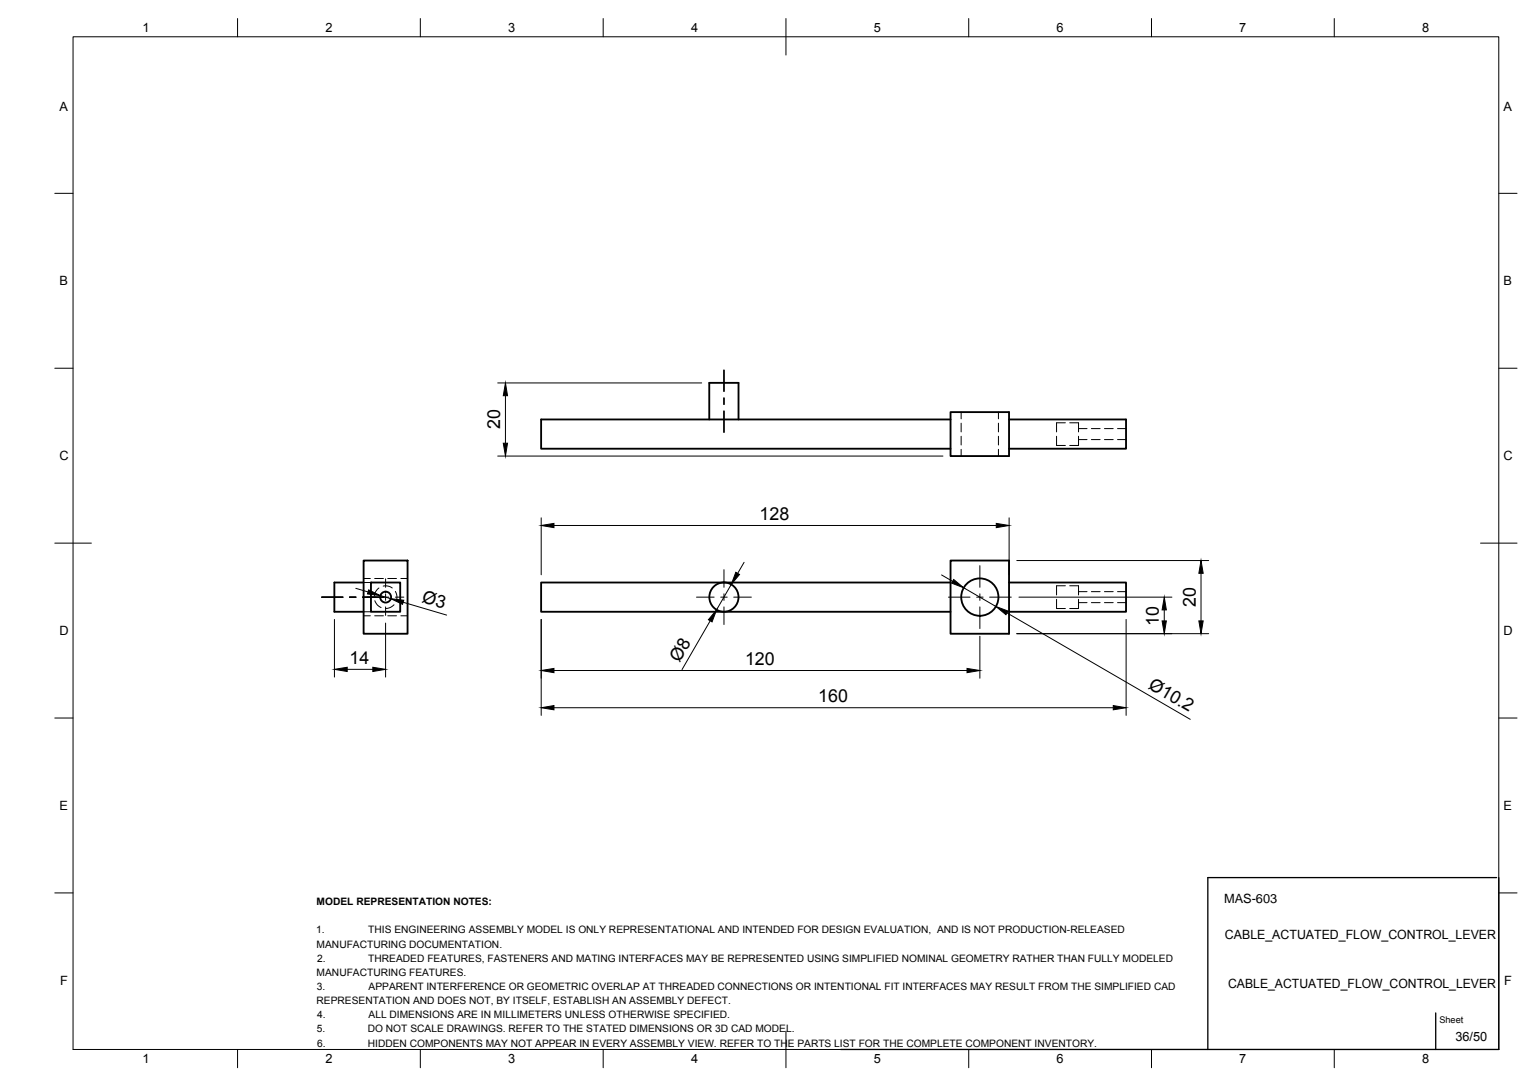
ISO-10303-21;
HEADER;
FILE_DESCRIPTION((''),'2;1');
FILE_NAME('CABLE_ACTUATED_FLOW_CONTROL_LEVER.step','2026-10-01T22:06:14-07:00',(''),(''),'','','');
FILE_SCHEMA (('AUTOMOTIVE_DESIGN { 1 0 10303 214 3 1 1 }'));
ENDSEC;
DATA;
#10=MECHANICAL_DESIGN_GEOMETRIC_PRESENTATION_REPRESENTATION('',(#1009),#50440);
#916=SHAPE_REPRESENTATION_RELATIONSHIP('SRR','None',#50649,#961) ;
#961=ADVANCED_BREP_SHAPE_REPRESENTATION('',(#1064),#50418) ;
#1009=STYLED_ITEM('',(#50883),#1064) ;
#1064=MANIFOLD_SOLID_BREP('CABLE_ACTUATED_FLOW_CONTROL_LEVER',#28676) ;
#1370=FACE_BOUND('',#5206,.T.) ;
#1371=FACE_BOUND('',#5211,.T.) ;
#1372=FACE_BOUND('',#5213,.T.) ;
#1373=FACE_BOUND('',#5215,.T.) ;
#1374=FACE_BOUND('',#5218,.T.) ;
#1375=FACE_BOUND('',#5229,.T.) ;
#2208=PLANE('',#30896) ;
#2209=PLANE('',#30897) ;
#2210=PLANE('',#30898) ;
#2211=PLANE('',#30902) ;
#2212=PLANE('',#30904) ;
#2213=PLANE('',#30910) ;
#2214=PLANE('',#30911) ;
#2215=PLANE('',#30912) ;
#2216=PLANE('',#30913) ;
#2217=PLANE('',#30914) ;
#2218=PLANE('',#30915) ;
#2219=PLANE('',#30916) ;
#2220=PLANE('',#30917) ;
#2221=PLANE('',#30918) ;
#2222=PLANE('',#30919) ;
#2223=PLANE('',#30920) ;
#2224=PLANE('',#30921) ;
#2225=PLANE('',#30922) ;
#2226=PLANE('',#30923) ;
#2227=PLANE('',#30924) ;
#3388=FACE_OUTER_BOUND('',#5200,.T.) ;
#3389=FACE_OUTER_BOUND('',#5201,.T.) ;
#3390=FACE_OUTER_BOUND('',#5202,.T.) ;
#3391=FACE_OUTER_BOUND('',#5203,.T.) ;
#3392=FACE_OUTER_BOUND('',#5204,.T.) ;
#3393=FACE_OUTER_BOUND('',#5205,.T.) ;
#3394=FACE_OUTER_BOUND('',#5207,.T.) ;
#3395=FACE_OUTER_BOUND('',#5208,.T.) ;
#3396=FACE_OUTER_BOUND('',#5209,.T.) ;
#3397=FACE_OUTER_BOUND('',#5210,.T.) ;
#3398=FACE_OUTER_BOUND('',#5212,.T.) ;
#3399=FACE_OUTER_BOUND('',#5214,.T.) ;
#3400=FACE_OUTER_BOUND('',#5216,.T.) ;
#3401=FACE_OUTER_BOUND('',#5217,.T.) ;
#3402=FACE_OUTER_BOUND('',#5219,.T.) ;
#3403=FACE_OUTER_BOUND('',#5220,.T.) ;
#3404=FACE_OUTER_BOUND('',#5221,.T.) ;
#3405=FACE_OUTER_BOUND('',#5222,.T.) ;
#3406=FACE_OUTER_BOUND('',#5223,.T.) ;
#3407=FACE_OUTER_BOUND('',#5224,.T.) ;
#3408=FACE_OUTER_BOUND('',#5225,.T.) ;
#3409=FACE_OUTER_BOUND('',#5226,.T.) ;
#3410=FACE_OUTER_BOUND('',#5227,.T.) ;
#3411=FACE_OUTER_BOUND('',#5228,.T.) ;
#5200=EDGE_LOOP('',(#23983,#23984,#23985,#23986,#23987)) ;
#5201=EDGE_LOOP('',(#23988)) ;
#5202=EDGE_LOOP('',(#23989,#23990,#23991,#23992)) ;
#5203=EDGE_LOOP('',(#23993,#23994,#23995,#23996)) ;
#5204=EDGE_LOOP('',(#23997,#23998,#23999,#24000)) ;
#5205=EDGE_LOOP('',(#24001)) ;
#5206=EDGE_LOOP('',(#24002)) ;
#5207=EDGE_LOOP('',(#24003)) ;
#5208=EDGE_LOOP('',(#24004,#24005,#24006,#24007)) ;
#5209=EDGE_LOOP('',(#24008,#24009,#24010,#24011)) ;
#5210=EDGE_LOOP('',(#24012,#24013,#24014,#24015)) ;
#5211=EDGE_LOOP('',(#24016,#24017,#24018,#24019)) ;
#5212=EDGE_LOOP('',(#24020,#24021,#24022,#24023)) ;
#5213=EDGE_LOOP('',(#24024,#24025,#24026,#24027)) ;
#5214=EDGE_LOOP('',(#24028,#24029,#24030,#24031)) ;
#5215=EDGE_LOOP('',(#24032)) ;
#5216=EDGE_LOOP('',(#24033,#24034,#24035,#24036)) ;
#5217=EDGE_LOOP('',(#24037,#24038,#24039,#24040)) ;
#5218=EDGE_LOOP('',(#24041)) ;
#5219=EDGE_LOOP('',(#24042,#24043,#24044,#24045)) ;
#5220=EDGE_LOOP('',(#24046,#24047,#24048,#24049,#24050)) ;
#5221=EDGE_LOOP('',(#24051,#24052,#24053,#24054,#24055)) ;
#5222=EDGE_LOOP('',(#24056,#24057,#24058,#24059)) ;
#5223=EDGE_LOOP('',(#24060,#24061,#24062,#24063)) ;
#5224=EDGE_LOOP('',(#24064,#24065,#24066,#24067)) ;
#5225=EDGE_LOOP('',(#24068,#24069,#24070,#24071)) ;
#5226=EDGE_LOOP('',(#24072,#24073,#24074,#24075)) ;
#5227=EDGE_LOOP('',(#24076,#24077,#24078,#24079)) ;
#5228=EDGE_LOOP('',(#24080,#24081,#24082,#24083)) ;
#5229=EDGE_LOOP('',(#24084)) ;
#7836=LINE('',#47072,#10308) ;
#7837=LINE('',#47077,#10309) ;
#7838=LINE('',#47079,#10310) ;
#7839=LINE('',#47080,#10311) ;
#7840=LINE('',#47083,#10312) ;
#7841=LINE('',#47085,#10313) ;
#7842=LINE('',#47086,#10314) ;
#7843=LINE('',#47091,#10315) ;
#7844=LINE('',#47100,#10316) ;
#7845=LINE('',#47105,#10317) ;
#7846=LINE('',#47110,#10318) ;
#7847=LINE('',#47112,#10319) ;
#7848=LINE('',#47114,#10320) ;
#7849=LINE('',#47115,#10321) ;
#7850=LINE('',#47118,#10322) ;
#7851=LINE('',#47120,#10323) ;
#7852=LINE('',#47122,#10324) ;
#7853=LINE('',#47123,#10325) ;
#7854=LINE('',#47127,#10326) ;
#7855=LINE('',#47129,#10327) ;
#7856=LINE('',#47131,#10328) ;
#7857=LINE('',#47132,#10329) ;
#7858=LINE('',#47134,#10330) ;
#7859=LINE('',#47136,#10331) ;
#7860=LINE('',#47137,#10332) ;
#7861=LINE('',#47139,#10333) ;
#7862=LINE('',#47140,#10334) ;
#7863=LINE('',#47142,#10335) ;
#7864=LINE('',#47144,#10336) ;
#7865=LINE('',#47148,#10337) ;
#7866=LINE('',#47149,#10338) ;
#7867=LINE('',#47152,#10339) ;
#7868=LINE('',#47153,#10340) ;
#7869=LINE('',#47155,#10341) ;
#7870=LINE('',#47159,#10342) ;
#7871=LINE('',#47161,#10343) ;
#7872=LINE('',#47162,#10344) ;
#7873=LINE('',#47165,#10345) ;
#7874=LINE('',#47166,#10346) ;
#7875=LINE('',#47169,#10347) ;
#7876=LINE('',#47170,#10348) ;
#7877=LINE('',#47172,#10349) ;
#10308=VECTOR('',#37851,0.4) ;
#10309=VECTOR('',#37858,1.) ;
#10310=VECTOR('',#37859,1.) ;
#10311=VECTOR('',#37860,1.) ;
#10312=VECTOR('',#37863,1.) ;
#10313=VECTOR('',#37864,1.) ;
#10314=VECTOR('',#37865,1.) ;
#10315=VECTOR('',#37870,0.31) ;
#10316=VECTOR('',#37883,0.15) ;
#10317=VECTOR('',#37888,0.51) ;
#10318=VECTOR('',#37893,1.) ;
#10319=VECTOR('',#37894,1.) ;
#10320=VECTOR('',#37895,1.) ;
#10321=VECTOR('',#37896,1.) ;
#10322=VECTOR('',#37897,1.) ;
#10323=VECTOR('',#37898,1.) ;
#10324=VECTOR('',#37899,1.) ;
#10325=VECTOR('',#37900,1.) ;
#10326=VECTOR('',#37903,1.) ;
#10327=VECTOR('',#37904,1.) ;
#10328=VECTOR('',#37905,1.) ;
#10329=VECTOR('',#37906,1.) ;
#10330=VECTOR('',#37907,1.) ;
#10331=VECTOR('',#37908,1.) ;
#10332=VECTOR('',#37909,1.) ;
#10333=VECTOR('',#37912,1.) ;
#10334=VECTOR('',#37913,1.) ;
#10335=VECTOR('',#37916,1.) ;
#10336=VECTOR('',#37919,1.) ;
#10337=VECTOR('',#37924,1.) ;
#10338=VECTOR('',#37925,1.) ;
#10339=VECTOR('',#37928,1.) ;
#10340=VECTOR('',#37929,1.) ;
#10341=VECTOR('',#37932,1.) ;
#10342=VECTOR('',#37937,1.) ;
#10343=VECTOR('',#37938,1.) ;
#10344=VECTOR('',#37939,1.) ;
#10345=VECTOR('',#37942,1.) ;
#10346=VECTOR('',#37943,1.) ;
#10347=VECTOR('',#37946,1.) ;
#10348=VECTOR('',#37947,1.) ;
#10349=VECTOR('',#37950,1.) ;
#11223=CIRCLE('',#30893,0.4) ;
#11224=CIRCLE('',#30894,0.4) ;
#11225=CIRCLE('',#30895,0.4) ;
#11226=CIRCLE('',#30900,0.31) ;
#11227=CIRCLE('',#30901,0.31) ;
#11228=CIRCLE('',#30903,0.15) ;
#11229=CIRCLE('',#30906,0.15) ;
#11230=CIRCLE('',#30908,0.51) ;
#11231=CIRCLE('',#30909,0.51) ;
#13643=VERTEX_POINT('',#47067) ;
#13644=VERTEX_POINT('',#47068) ;
#13645=VERTEX_POINT('',#47071) ;
#13646=VERTEX_POINT('',#47076) ;
#13647=VERTEX_POINT('',#47078) ;
#13648=VERTEX_POINT('',#47082) ;
#13649=VERTEX_POINT('',#47084) ;
#13650=VERTEX_POINT('',#47088) ;
#13651=VERTEX_POINT('',#47090) ;
#13652=VERTEX_POINT('',#47094) ;
#13653=VERTEX_POINT('',#47098) ;
#13654=VERTEX_POINT('',#47102) ;
#13655=VERTEX_POINT('',#47104) ;
#13656=VERTEX_POINT('',#47108) ;
#13657=VERTEX_POINT('',#47109) ;
#13658=VERTEX_POINT('',#47111) ;
#13659=VERTEX_POINT('',#47113) ;
#13660=VERTEX_POINT('',#47116) ;
#13661=VERTEX_POINT('',#47117) ;
#13662=VERTEX_POINT('',#47119) ;
#13663=VERTEX_POINT('',#47121) ;
#13664=VERTEX_POINT('',#47125) ;
#13665=VERTEX_POINT('',#47126) ;
#13666=VERTEX_POINT('',#47128) ;
#13667=VERTEX_POINT('',#47130) ;
#13668=VERTEX_POINT('',#47133) ;
#13669=VERTEX_POINT('',#47135) ;
#13670=VERTEX_POINT('',#47147) ;
#13671=VERTEX_POINT('',#47151) ;
#13672=VERTEX_POINT('',#47158) ;
#13673=VERTEX_POINT('',#47160) ;
#13674=VERTEX_POINT('',#47164) ;
#13675=VERTEX_POINT('',#47168) ;
#17257=EDGE_CURVE('',#13643,#13644,#11223,.T.) ;
#17258=EDGE_CURVE('',#13644,#13643,#11224,.T.) ;
#17259=EDGE_CURVE('',#13644,#13645,#7836,.T.) ;
#17260=EDGE_CURVE('',#13645,#13645,#11225,.T.) ;
#17261=EDGE_CURVE('',#13646,#13643,#7837,.T.) ;
#17262=EDGE_CURVE('',#13647,#13646,#7838,.T.) ;
#17263=EDGE_CURVE('',#13647,#13644,#7839,.T.) ;
#17264=EDGE_CURVE('',#13644,#13648,#7840,.T.) ;
#17265=EDGE_CURVE('',#13648,#13649,#7841,.T.) ;
#17266=EDGE_CURVE('',#13643,#13649,#7842,.T.) ;
#17267=EDGE_CURVE('',#13650,#13650,#11226,.T.) ;
#17268=EDGE_CURVE('',#13650,#13651,#7843,.T.) ;
#17269=EDGE_CURVE('',#13651,#13651,#11227,.T.) ;
#17270=EDGE_CURVE('',#13652,#13652,#11228,.T.) ;
#17271=EDGE_CURVE('',#13653,#13653,#11229,.T.) ;
#17272=EDGE_CURVE('',#13653,#13652,#7844,.T.) ;
#17273=EDGE_CURVE('',#13654,#13654,#11230,.T.) ;
#17274=EDGE_CURVE('',#13654,#13655,#7845,.T.) ;
#17275=EDGE_CURVE('',#13655,#13655,#11231,.T.) ;
#17276=EDGE_CURVE('',#13656,#13657,#7846,.T.) ;
#17277=EDGE_CURVE('',#13657,#13658,#7847,.T.) ;
#17278=EDGE_CURVE('',#13658,#13659,#7848,.T.) ;
#17279=EDGE_CURVE('',#13659,#13656,#7849,.T.) ;
#17280=EDGE_CURVE('',#13660,#13661,#7850,.T.) ;
#17281=EDGE_CURVE('',#13662,#13660,#7851,.T.) ;
#17282=EDGE_CURVE('',#13663,#13662,#7852,.T.) ;
#17283=EDGE_CURVE('',#13661,#13663,#7853,.T.) ;
#17284=EDGE_CURVE('',#13664,#13665,#7854,.T.) ;
#17285=EDGE_CURVE('',#13665,#13666,#7855,.T.) ;
#17286=EDGE_CURVE('',#13666,#13667,#7856,.T.) ;
#17287=EDGE_CURVE('',#13667,#13664,#7857,.T.) ;
#17288=EDGE_CURVE('',#13649,#13668,#7858,.T.) ;
#17289=EDGE_CURVE('',#13669,#13648,#7859,.T.) ;
#17290=EDGE_CURVE('',#13668,#13669,#7860,.T.) ;
#17291=EDGE_CURVE('',#13667,#13658,#7861,.T.) ;
#17292=EDGE_CURVE('',#13664,#13657,#7862,.T.) ;
#17293=EDGE_CURVE('',#13666,#13659,#7863,.T.) ;
#17294=EDGE_CURVE('',#13665,#13656,#7864,.T.) ;
#17295=EDGE_CURVE('',#13670,#13647,#7865,.T.) ;
#17296=EDGE_CURVE('',#13670,#13669,#7866,.T.) ;
#17297=EDGE_CURVE('',#13671,#13668,#7867,.T.) ;
#17298=EDGE_CURVE('',#13646,#13671,#7868,.T.) ;
#17299=EDGE_CURVE('',#13671,#13670,#7869,.T.) ;
#17300=EDGE_CURVE('',#13662,#13672,#7870,.T.) ;
#17301=EDGE_CURVE('',#13673,#13672,#7871,.T.) ;
#17302=EDGE_CURVE('',#13663,#13673,#7872,.T.) ;
#17303=EDGE_CURVE('',#13660,#13674,#7873,.T.) ;
#17304=EDGE_CURVE('',#13672,#13674,#7874,.T.) ;
#17305=EDGE_CURVE('',#13661,#13675,#7875,.T.) ;
#17306=EDGE_CURVE('',#13674,#13675,#7876,.T.) ;
#17307=EDGE_CURVE('',#13675,#13673,#7877,.T.) ;
#23983=ORIENTED_EDGE('',*,*,#17257,.F.) ;
#23984=ORIENTED_EDGE('',*,*,#17258,.F.) ;
#23985=ORIENTED_EDGE('',*,*,#17259,.T.) ;
#23986=ORIENTED_EDGE('',*,*,#17260,.F.) ;
#23987=ORIENTED_EDGE('',*,*,#17259,.F.) ;
#23988=ORIENTED_EDGE('',*,*,#17260,.T.) ;
#23989=ORIENTED_EDGE('',*,*,#17258,.T.) ;
#23990=ORIENTED_EDGE('',*,*,#17261,.F.) ;
#23991=ORIENTED_EDGE('',*,*,#17262,.F.) ;
#23992=ORIENTED_EDGE('',*,*,#17263,.T.) ;
#23993=ORIENTED_EDGE('',*,*,#17257,.T.) ;
#23994=ORIENTED_EDGE('',*,*,#17264,.T.) ;
#23995=ORIENTED_EDGE('',*,*,#17265,.T.) ;
#23996=ORIENTED_EDGE('',*,*,#17266,.F.) ;
#23997=ORIENTED_EDGE('',*,*,#17267,.T.) ;
#23998=ORIENTED_EDGE('',*,*,#17268,.T.) ;
#23999=ORIENTED_EDGE('',*,*,#17269,.T.) ;
#24000=ORIENTED_EDGE('',*,*,#17268,.F.) ;
#24001=ORIENTED_EDGE('',*,*,#17267,.F.) ;
#24002=ORIENTED_EDGE('',*,*,#17270,.F.) ;
#24003=ORIENTED_EDGE('',*,*,#17269,.F.) ;
#24004=ORIENTED_EDGE('',*,*,#17271,.F.) ;
#24005=ORIENTED_EDGE('',*,*,#17272,.T.) ;
#24006=ORIENTED_EDGE('',*,*,#17270,.T.) ;
#24007=ORIENTED_EDGE('',*,*,#17272,.F.) ;
#24008=ORIENTED_EDGE('',*,*,#17273,.F.) ;
#24009=ORIENTED_EDGE('',*,*,#17274,.T.) ;
#24010=ORIENTED_EDGE('',*,*,#17275,.F.) ;
#24011=ORIENTED_EDGE('',*,*,#17274,.F.) ;
#24012=ORIENTED_EDGE('',*,*,#17276,.T.) ;
#24013=ORIENTED_EDGE('',*,*,#17277,.T.) ;
#24014=ORIENTED_EDGE('',*,*,#17278,.T.) ;
#24015=ORIENTED_EDGE('',*,*,#17279,.T.) ;
#24016=ORIENTED_EDGE('',*,*,#17280,.F.) ;
#24017=ORIENTED_EDGE('',*,*,#17281,.F.) ;
#24018=ORIENTED_EDGE('',*,*,#17282,.F.) ;
#24019=ORIENTED_EDGE('',*,*,#17283,.F.) ;
#24020=ORIENTED_EDGE('',*,*,#17284,.T.) ;
#24021=ORIENTED_EDGE('',*,*,#17285,.T.) ;
#24022=ORIENTED_EDGE('',*,*,#17286,.T.) ;
#24023=ORIENTED_EDGE('',*,*,#17287,.T.) ;
#24024=ORIENTED_EDGE('',*,*,#17288,.F.) ;
#24025=ORIENTED_EDGE('',*,*,#17265,.F.) ;
#24026=ORIENTED_EDGE('',*,*,#17289,.F.) ;
#24027=ORIENTED_EDGE('',*,*,#17290,.F.) ;
#24028=ORIENTED_EDGE('',*,*,#17291,.T.) ;
#24029=ORIENTED_EDGE('',*,*,#17277,.F.) ;
#24030=ORIENTED_EDGE('',*,*,#17292,.F.) ;
#24031=ORIENTED_EDGE('',*,*,#17287,.F.) ;
#24032=ORIENTED_EDGE('',*,*,#17273,.T.) ;
#24033=ORIENTED_EDGE('',*,*,#17293,.T.) ;
#24034=ORIENTED_EDGE('',*,*,#17278,.F.) ;
#24035=ORIENTED_EDGE('',*,*,#17291,.F.) ;
#24036=ORIENTED_EDGE('',*,*,#17286,.F.) ;
#24037=ORIENTED_EDGE('',*,*,#17294,.T.) ;
#24038=ORIENTED_EDGE('',*,*,#17279,.F.) ;
#24039=ORIENTED_EDGE('',*,*,#17293,.F.) ;
#24040=ORIENTED_EDGE('',*,*,#17285,.F.) ;
#24041=ORIENTED_EDGE('',*,*,#17275,.T.) ;
#24042=ORIENTED_EDGE('',*,*,#17292,.T.) ;
#24043=ORIENTED_EDGE('',*,*,#17276,.F.) ;
#24044=ORIENTED_EDGE('',*,*,#17294,.F.) ;
#24045=ORIENTED_EDGE('',*,*,#17284,.F.) ;
#24046=ORIENTED_EDGE('',*,*,#17289,.T.) ;
#24047=ORIENTED_EDGE('',*,*,#17264,.F.) ;
#24048=ORIENTED_EDGE('',*,*,#17263,.F.) ;
#24049=ORIENTED_EDGE('',*,*,#17295,.F.) ;
#24050=ORIENTED_EDGE('',*,*,#17296,.T.) ;
#24051=ORIENTED_EDGE('',*,*,#17288,.T.) ;
#24052=ORIENTED_EDGE('',*,*,#17297,.F.) ;
#24053=ORIENTED_EDGE('',*,*,#17298,.F.) ;
#24054=ORIENTED_EDGE('',*,*,#17261,.T.) ;
#24055=ORIENTED_EDGE('',*,*,#17266,.T.) ;
#24056=ORIENTED_EDGE('',*,*,#17298,.T.) ;
#24057=ORIENTED_EDGE('',*,*,#17299,.T.) ;
#24058=ORIENTED_EDGE('',*,*,#17295,.T.) ;
#24059=ORIENTED_EDGE('',*,*,#17262,.T.) ;
#24060=ORIENTED_EDGE('',*,*,#17290,.T.) ;
#24061=ORIENTED_EDGE('',*,*,#17296,.F.) ;
#24062=ORIENTED_EDGE('',*,*,#17299,.F.) ;
#24063=ORIENTED_EDGE('',*,*,#17297,.T.) ;
#24064=ORIENTED_EDGE('',*,*,#17282,.T.) ;
#24065=ORIENTED_EDGE('',*,*,#17300,.T.) ;
#24066=ORIENTED_EDGE('',*,*,#17301,.F.) ;
#24067=ORIENTED_EDGE('',*,*,#17302,.F.) ;
#24068=ORIENTED_EDGE('',*,*,#17281,.T.) ;
#24069=ORIENTED_EDGE('',*,*,#17303,.T.) ;
#24070=ORIENTED_EDGE('',*,*,#17304,.F.) ;
#24071=ORIENTED_EDGE('',*,*,#17300,.F.) ;
#24072=ORIENTED_EDGE('',*,*,#17280,.T.) ;
#24073=ORIENTED_EDGE('',*,*,#17305,.T.) ;
#24074=ORIENTED_EDGE('',*,*,#17306,.F.) ;
#24075=ORIENTED_EDGE('',*,*,#17303,.F.) ;
#24076=ORIENTED_EDGE('',*,*,#17283,.T.) ;
#24077=ORIENTED_EDGE('',*,*,#17302,.T.) ;
#24078=ORIENTED_EDGE('',*,*,#17307,.F.) ;
#24079=ORIENTED_EDGE('',*,*,#17305,.F.) ;
#24080=ORIENTED_EDGE('',*,*,#17307,.T.) ;
#24081=ORIENTED_EDGE('',*,*,#17301,.T.) ;
#24082=ORIENTED_EDGE('',*,*,#17304,.T.) ;
#24083=ORIENTED_EDGE('',*,*,#17306,.T.) ;
#24084=ORIENTED_EDGE('',*,*,#17271,.T.) ;
#26865=CYLINDRICAL_SURFACE('',#30892,0.4) ;
#26866=CYLINDRICAL_SURFACE('',#30899,0.31) ;
#26867=CYLINDRICAL_SURFACE('',#30905,0.15) ;
#26868=CYLINDRICAL_SURFACE('',#30907,0.51) ;
#28123=ADVANCED_FACE('',(#3388),#26865,.T.) ;
#28124=ADVANCED_FACE('',(#3389),#2208,.T.) ;
#28125=ADVANCED_FACE('',(#3390),#2209,.F.) ;
#28126=ADVANCED_FACE('',(#3391),#2210,.F.) ;
#28127=ADVANCED_FACE('',(#3392),#26866,.F.) ;
#28128=ADVANCED_FACE('',(#3393,#1370),#2211,.F.) ;
#28129=ADVANCED_FACE('',(#3394),#2212,.F.) ;
#28130=ADVANCED_FACE('',(#3395),#26867,.F.) ;
#28131=ADVANCED_FACE('',(#3396),#26868,.F.) ;
#28132=ADVANCED_FACE('',(#3397,#1371),#2213,.F.) ;
#28133=ADVANCED_FACE('',(#3398,#1372),#2214,.T.) ;
#28134=ADVANCED_FACE('',(#3399,#1373),#2215,.F.) ;
#28135=ADVANCED_FACE('',(#3400),#2216,.F.) ;
#28136=ADVANCED_FACE('',(#3401,#1374),#2217,.F.) ;
#28137=ADVANCED_FACE('',(#3402),#2218,.F.) ;
#28138=ADVANCED_FACE('',(#3403),#2219,.F.) ;
#28139=ADVANCED_FACE('',(#3404),#2220,.F.) ;
#28140=ADVANCED_FACE('',(#3405),#2221,.T.) ;
#28141=ADVANCED_FACE('',(#3406),#2222,.F.) ;
#28142=ADVANCED_FACE('',(#3407),#2223,.F.) ;
#28143=ADVANCED_FACE('',(#3408),#2224,.F.) ;
#28144=ADVANCED_FACE('',(#3409),#2225,.F.) ;
#28145=ADVANCED_FACE('',(#3410),#2226,.F.) ;
#28146=ADVANCED_FACE('',(#3411,#1375),#2227,.F.) ;
#28676=CLOSED_SHELL('',(#28123,#28124,#28125,#28126,#28127,#28128,#28129,
#28130,#28131,#28132,#28133,#28134,#28135,#28136,#28137,#28138,#28139,#28140,
#28141,#28142,#28143,#28144,#28145,#28146)) ;
#30891=AXIS2_PLACEMENT_3D('',#47065,#37843,#37844) ;
#30892=AXIS2_PLACEMENT_3D('',#47066,#37845,#37846) ;
#30893=AXIS2_PLACEMENT_3D('',#47069,#37847,#37848) ;
#30894=AXIS2_PLACEMENT_3D('',#47070,#37849,#37850) ;
#30895=AXIS2_PLACEMENT_3D('',#47073,#37852,#37853) ;
#30896=AXIS2_PLACEMENT_3D('',#47074,#37854,#37855) ;
#30897=AXIS2_PLACEMENT_3D('',#47075,#37856,#37857) ;
#30898=AXIS2_PLACEMENT_3D('',#47081,#37861,#37862) ;
#30899=AXIS2_PLACEMENT_3D('',#47087,#37866,#37867) ;
#30900=AXIS2_PLACEMENT_3D('',#47089,#37868,#37869) ;
#30901=AXIS2_PLACEMENT_3D('',#47092,#37871,#37872) ;
#30902=AXIS2_PLACEMENT_3D('',#47093,#37873,#37874) ;
#30903=AXIS2_PLACEMENT_3D('',#47095,#37875,#37876) ;
#30904=AXIS2_PLACEMENT_3D('',#47096,#37877,#37878) ;
#30905=AXIS2_PLACEMENT_3D('',#47097,#37879,#37880) ;
#30906=AXIS2_PLACEMENT_3D('',#47099,#37881,#37882) ;
#30907=AXIS2_PLACEMENT_3D('',#47101,#37884,#37885) ;
#30908=AXIS2_PLACEMENT_3D('',#47103,#37886,#37887) ;
#30909=AXIS2_PLACEMENT_3D('',#47106,#37889,#37890) ;
#30910=AXIS2_PLACEMENT_3D('',#47107,#37891,#37892) ;
#30911=AXIS2_PLACEMENT_3D('',#47124,#37901,#37902) ;
#30912=AXIS2_PLACEMENT_3D('',#47138,#37910,#37911) ;
#30913=AXIS2_PLACEMENT_3D('',#47141,#37914,#37915) ;
#30914=AXIS2_PLACEMENT_3D('',#47143,#37917,#37918) ;
#30915=AXIS2_PLACEMENT_3D('',#47145,#37920,#37921) ;
#30916=AXIS2_PLACEMENT_3D('',#47146,#37922,#37923) ;
#30917=AXIS2_PLACEMENT_3D('',#47150,#37926,#37927) ;
#30918=AXIS2_PLACEMENT_3D('',#47154,#37930,#37931) ;
#30919=AXIS2_PLACEMENT_3D('',#47156,#37933,#37934) ;
#30920=AXIS2_PLACEMENT_3D('',#47157,#37935,#37936) ;
#30921=AXIS2_PLACEMENT_3D('',#47163,#37940,#37941) ;
#30922=AXIS2_PLACEMENT_3D('',#47167,#37944,#37945) ;
#30923=AXIS2_PLACEMENT_3D('',#47171,#37948,#37949) ;
#30924=AXIS2_PLACEMENT_3D('',#47173,#37951,#37952) ;
#37843=DIRECTION('axis',(0.,0.,1.)) ;
#37844=DIRECTION('refdir',(1.,0.,0.)) ;
#37845=DIRECTION('center_axis',(0.,1.,0.)) ;
#37846=DIRECTION('ref_axis',(1.,0.,0.)) ;
#37847=DIRECTION('center_axis',(0.,1.,0.)) ;
#37848=DIRECTION('ref_axis',(1.,0.,0.)) ;
#37849=DIRECTION('center_axis',(0.,1.,0.)) ;
#37850=DIRECTION('ref_axis',(1.,0.,0.)) ;
#37851=DIRECTION('',(0.,-1.,0.)) ;
#37852=DIRECTION('center_axis',(0.,-1.,0.)) ;
#37853=DIRECTION('ref_axis',(1.,0.,0.)) ;
#37854=DIRECTION('center_axis',(0.,-1.,0.)) ;
#37855=DIRECTION('ref_axis',(-1.,0.,0.)) ;
#37856=DIRECTION('center_axis',(0.,1.,0.)) ;
#37857=DIRECTION('ref_axis',(0.,0.,1.)) ;
#37858=DIRECTION('',(0.,0.,-1.)) ;
#37859=DIRECTION('',(1.,0.,0.)) ;
#37860=DIRECTION('',(0.,0.,-1.)) ;
#37861=DIRECTION('center_axis',(0.,1.,0.)) ;
#37862=DIRECTION('ref_axis',(0.,0.,1.)) ;
#37863=DIRECTION('',(0.,0.,-1.)) ;
#37864=DIRECTION('',(1.,0.,0.)) ;
#37865=DIRECTION('',(0.,0.,-1.)) ;
#37866=DIRECTION('center_axis',(0.,0.,1.)) ;
#37867=DIRECTION('ref_axis',(1.,0.,0.)) ;
#37868=DIRECTION('center_axis',(0.,0.,-1.)) ;
#37869=DIRECTION('ref_axis',(1.,0.,0.)) ;
#37870=DIRECTION('',(0.,0.,1.)) ;
#37871=DIRECTION('center_axis',(0.,0.,1.)) ;
#37872=DIRECTION('ref_axis',(1.,0.,0.)) ;
#37873=DIRECTION('center_axis',(0.,0.,-1.)) ;
#37874=DIRECTION('ref_axis',(-1.,0.,0.)) ;
#37875=DIRECTION('center_axis',(0.,0.,1.)) ;
#37876=DIRECTION('ref_axis',(1.,0.,0.)) ;
#37877=DIRECTION('center_axis',(0.,0.,1.)) ;
#37878=DIRECTION('ref_axis',(1.,0.,0.)) ;
#37879=DIRECTION('center_axis',(0.,0.,1.)) ;
#37880=DIRECTION('ref_axis',(1.,0.,0.)) ;
#37881=DIRECTION('center_axis',(0.,0.,1.)) ;
#37882=DIRECTION('ref_axis',(1.,0.,0.)) ;
#37883=DIRECTION('',(0.,0.,1.)) ;
#37884=DIRECTION('center_axis',(0.,1.,0.)) ;
#37885=DIRECTION('ref_axis',(1.,0.,0.)) ;
#37886=DIRECTION('center_axis',(0.,1.,0.)) ;
#37887=DIRECTION('ref_axis',(1.,0.,0.)) ;
#37888=DIRECTION('',(0.,1.,0.)) ;
#37889=DIRECTION('center_axis',(0.,-1.,0.)) ;
#37890=DIRECTION('ref_axis',(1.,0.,0.)) ;
#37891=DIRECTION('center_axis',(0.,0.,1.)) ;
#37892=DIRECTION('ref_axis',(1.,0.,0.)) ;
#37893=DIRECTION('',(0.,-1.,0.)) ;
#37894=DIRECTION('',(-1.,0.,0.)) ;
#37895=DIRECTION('',(0.,1.,0.)) ;
#37896=DIRECTION('',(1.,0.,0.)) ;
#37897=DIRECTION('',(1.,0.,0.)) ;
#37898=DIRECTION('',(0.,1.,0.)) ;
#37899=DIRECTION('',(-1.,0.,0.)) ;
#37900=DIRECTION('',(0.,-1.,0.)) ;
#37901=DIRECTION('center_axis',(0.,0.,1.)) ;
#37902=DIRECTION('ref_axis',(1.,0.,0.)) ;
#37903=DIRECTION('',(0.,1.,0.)) ;
#37904=DIRECTION('',(-1.,0.,0.)) ;
#37905=DIRECTION('',(0.,-1.,0.)) ;
#37906=DIRECTION('',(1.,0.,0.)) ;
#37907=DIRECTION('',(0.,1.,0.)) ;
#37908=DIRECTION('',(0.,-1.,0.)) ;
#37909=DIRECTION('',(-1.,0.,0.)) ;
#37910=DIRECTION('center_axis',(0.,1.,0.)) ;
#37911=DIRECTION('ref_axis',(0.,0.,1.)) ;
#37912=DIRECTION('',(0.,0.,-1.)) ;
#37913=DIRECTION('',(0.,0.,-1.)) ;
#37914=DIRECTION('center_axis',(1.,0.,0.)) ;
#37915=DIRECTION('ref_axis',(0.,0.,-1.)) ;
#37916=DIRECTION('',(0.,0.,-1.)) ;
#37917=DIRECTION('center_axis',(0.,-1.,0.)) ;
#37918=DIRECTION('ref_axis',(0.,0.,-1.)) ;
#37919=DIRECTION('',(0.,0.,-1.)) ;
#37920=DIRECTION('center_axis',(-1.,0.,0.)) ;
#37921=DIRECTION('ref_axis',(0.,0.,1.)) ;
#37922=DIRECTION('center_axis',(1.,0.,0.)) ;
#37923=DIRECTION('ref_axis',(0.,0.,-1.)) ;
#37924=DIRECTION('',(0.,-1.,0.)) ;
#37925=DIRECTION('',(0.,0.,-1.)) ;
#37926=DIRECTION('center_axis',(-1.,0.,0.)) ;
#37927=DIRECTION('ref_axis',(0.,0.,1.)) ;
#37928=DIRECTION('',(0.,0.,-1.)) ;
#37929=DIRECTION('',(0.,1.,0.)) ;
#37930=DIRECTION('center_axis',(0.,0.,1.)) ;
#37931=DIRECTION('ref_axis',(1.,0.,0.)) ;
#37932=DIRECTION('',(-1.,0.,0.)) ;
#37933=DIRECTION('center_axis',(0.,-1.,0.)) ;
#37934=DIRECTION('ref_axis',(0.,0.,-1.)) ;
#37935=DIRECTION('center_axis',(0.,1.,0.)) ;
#37936=DIRECTION('ref_axis',(0.,0.,1.)) ;
#37937=DIRECTION('',(0.,0.,-1.)) ;
#37938=DIRECTION('',(-1.,0.,0.)) ;
#37939=DIRECTION('',(0.,0.,-1.)) ;
#37940=DIRECTION('center_axis',(1.,0.,0.)) ;
#37941=DIRECTION('ref_axis',(0.,0.,-1.)) ;
#37942=DIRECTION('',(0.,0.,-1.)) ;
#37943=DIRECTION('',(0.,1.,0.)) ;
#37944=DIRECTION('center_axis',(0.,-1.,0.)) ;
#37945=DIRECTION('ref_axis',(0.,0.,-1.)) ;
#37946=DIRECTION('',(0.,0.,-1.)) ;
#37947=DIRECTION('',(1.,0.,0.)) ;
#37948=DIRECTION('center_axis',(-1.,0.,0.)) ;
#37949=DIRECTION('ref_axis',(0.,0.,1.)) ;
#37950=DIRECTION('',(0.,-1.,0.)) ;
#37951=DIRECTION('center_axis',(0.,0.,1.)) ;
#37952=DIRECTION('ref_axis',(1.,0.,0.)) ;
#47065=CARTESIAN_POINT('',(0.,0.,0.)) ;
#47066=CARTESIAN_POINT('Origin',(-53.,18.1,99.)) ;
#47067=CARTESIAN_POINT('',(-52.6,18.6,99.)) ;
#47068=CARTESIAN_POINT('',(-53.4,18.6,99.)) ;
#47069=CARTESIAN_POINT('Origin',(-53.,18.6,99.)) ;
#47070=CARTESIAN_POINT('Origin',(-53.,18.6,99.)) ;
#47071=CARTESIAN_POINT('',(-53.4,17.6,99.)) ;
#47072=CARTESIAN_POINT('',(-53.4,18.1,99.)) ;
#47073=CARTESIAN_POINT('Origin',(-53.,17.6,99.)) ;
#47074=CARTESIAN_POINT('Origin',(-53.,17.6,99.)) ;
#47075=CARTESIAN_POINT('Origin',(-53.,18.6,96.)) ;
#47076=CARTESIAN_POINT('',(-52.6,18.6,104.)) ;
#47077=CARTESIAN_POINT('',(-52.6,18.6,96.)) ;
#47078=CARTESIAN_POINT('',(-53.4,18.6,104.)) ;
#47079=CARTESIAN_POINT('',(-53.,18.6,104.)) ;
#47080=CARTESIAN_POINT('',(-53.4,18.6,96.)) ;
#47081=CARTESIAN_POINT('Origin',(-53.,18.6,96.)) ;
#47082=CARTESIAN_POINT('',(-53.4,18.6,92.8)) ;
#47083=CARTESIAN_POINT('',(-53.4,18.6,96.)) ;
#47084=CARTESIAN_POINT('',(-52.6,18.6,92.8)) ;
#47085=CARTESIAN_POINT('',(-53.,18.6,92.8)) ;
#47086=CARTESIAN_POINT('',(-52.6,18.6,96.)) ;
#47087=CARTESIAN_POINT('Origin',(-53.,19.,89.6)) ;
#47088=CARTESIAN_POINT('',(-53.31,19.,89.3)) ;
#47089=CARTESIAN_POINT('Origin',(-53.,19.,89.3)) ;
#47090=CARTESIAN_POINT('',(-53.31,19.,89.9)) ;
#47091=CARTESIAN_POINT('',(-53.31,19.,89.6)) ;
#47092=CARTESIAN_POINT('Origin',(-53.,19.,89.9)) ;
#47093=CARTESIAN_POINT('Origin',(-53.,19.,89.3)) ;
#47094=CARTESIAN_POINT('',(-53.15,19.,89.3)) ;
#47095=CARTESIAN_POINT('Origin',(-53.,19.,89.3)) ;
#47096=CARTESIAN_POINT('Origin',(-53.,19.,89.9)) ;
#47097=CARTESIAN_POINT('Origin',(-53.,19.,88.7)) ;
#47098=CARTESIAN_POINT('',(-53.15,19.,88.)) ;
#47099=CARTESIAN_POINT('Origin',(-53.,19.,88.)) ;
#47100=CARTESIAN_POINT('',(-53.15,19.,88.7)) ;
#47101=CARTESIAN_POINT('Origin',(-53.,19.,92.)) ;
#47102=CARTESIAN_POINT('',(-53.51,18.4,92.)) ;
#47103=CARTESIAN_POINT('Origin',(-53.,18.4,92.)) ;
#47104=CARTESIAN_POINT('',(-53.51,19.6,92.)) ;
#47105=CARTESIAN_POINT('',(-53.51,19.,92.)) ;
#47106=CARTESIAN_POINT('Origin',(-53.,19.6,92.)) ;
#47107=CARTESIAN_POINT('Origin',(-53.,19.,91.2)) ;
#47108=CARTESIAN_POINT('',(-52.,19.6,91.2)) ;
#47109=CARTESIAN_POINT('',(-52.,18.4,91.2)) ;
#47110=CARTESIAN_POINT('',(-52.,19.,91.2)) ;
#47111=CARTESIAN_POINT('',(-54.,18.4,91.2)) ;
#47112=CARTESIAN_POINT('',(-53.,18.4,91.2)) ;
#47113=CARTESIAN_POINT('',(-54.,19.6,91.2)) ;
#47114=CARTESIAN_POINT('',(-54.,19.,91.2)) ;
#47115=CARTESIAN_POINT('',(-53.,19.6,91.2)) ;
#47116=CARTESIAN_POINT('',(-53.4,19.4,91.2)) ;
#47117=CARTESIAN_POINT('',(-52.6,19.4,91.2)) ;
#47118=CARTESIAN_POINT('',(-53.,19.4,91.2)) ;
#47119=CARTESIAN_POINT('',(-53.4,18.6,91.2)) ;
#47120=CARTESIAN_POINT('',(-53.4,19.,91.2)) ;
#47121=CARTESIAN_POINT('',(-52.6,18.6,91.2)) ;
#47122=CARTESIAN_POINT('',(-53.,18.6,91.2)) ;
#47123=CARTESIAN_POINT('',(-52.6,19.,91.2)) ;
#47124=CARTESIAN_POINT('Origin',(-53.,19.,92.8)) ;
#47125=CARTESIAN_POINT('',(-52.,18.4,92.8)) ;
#47126=CARTESIAN_POINT('',(-52.,19.6,92.8)) ;
#47127=CARTESIAN_POINT('',(-52.,19.,92.8)) ;
#47128=CARTESIAN_POINT('',(-54.,19.6,92.8)) ;
#47129=CARTESIAN_POINT('',(-53.,19.6,92.8)) ;
#47130=CARTESIAN_POINT('',(-54.,18.4,92.8)) ;
#47131=CARTESIAN_POINT('',(-54.,19.,92.8)) ;
#47132=CARTESIAN_POINT('',(-53.,18.4,92.8)) ;
#47133=CARTESIAN_POINT('',(-52.6,19.4,92.8)) ;
#47134=CARTESIAN_POINT('',(-52.6,19.,92.8)) ;
#47135=CARTESIAN_POINT('',(-53.4,19.4,92.8)) ;
#47136=CARTESIAN_POINT('',(-53.4,19.,92.8)) ;
#47137=CARTESIAN_POINT('',(-53.,19.4,92.8)) ;
#47138=CARTESIAN_POINT('Origin',(-53.,18.4,92.)) ;
#47139=CARTESIAN_POINT('',(-54.,18.4,92.)) ;
#47140=CARTESIAN_POINT('',(-52.,18.4,92.)) ;
#47141=CARTESIAN_POINT('Origin',(-54.,19.,92.)) ;
#47142=CARTESIAN_POINT('',(-54.,19.6,92.)) ;
#47143=CARTESIAN_POINT('Origin',(-53.,19.6,92.)) ;
#47144=CARTESIAN_POINT('',(-52.,19.6,92.)) ;
#47145=CARTESIAN_POINT('Origin',(-52.,19.,92.)) ;
#47146=CARTESIAN_POINT('Origin',(-53.4,19.,96.)) ;
#47147=CARTESIAN_POINT('',(-53.4,19.4,104.)) ;
#47148=CARTESIAN_POINT('',(-53.4,19.,104.)) ;
#47149=CARTESIAN_POINT('',(-53.4,19.4,96.)) ;
#47150=CARTESIAN_POINT('Origin',(-52.6,19.,96.)) ;
#47151=CARTESIAN_POINT('',(-52.6,19.4,104.)) ;
#47152=CARTESIAN_POINT('',(-52.6,19.4,96.)) ;
#47153=CARTESIAN_POINT('',(-52.6,19.,104.)) ;
#47154=CARTESIAN_POINT('Origin',(-53.,19.,104.)) ;
#47155=CARTESIAN_POINT('',(-53.,19.4,104.)) ;
#47156=CARTESIAN_POINT('Origin',(-53.,19.4,96.)) ;
#47157=CARTESIAN_POINT('Origin',(-53.,18.6,96.)) ;
#47158=CARTESIAN_POINT('',(-53.4,18.6,88.)) ;
#47159=CARTESIAN_POINT('',(-53.4,18.6,96.)) ;
#47160=CARTESIAN_POINT('',(-52.6,18.6,88.)) ;
#47161=CARTESIAN_POINT('',(-53.,18.6,88.)) ;
#47162=CARTESIAN_POINT('',(-52.6,18.6,96.)) ;
#47163=CARTESIAN_POINT('Origin',(-53.4,19.,96.)) ;
#47164=CARTESIAN_POINT('',(-53.4,19.4,88.)) ;
#47165=CARTESIAN_POINT('',(-53.4,19.4,96.)) ;
#47166=CARTESIAN_POINT('',(-53.4,19.,88.)) ;
#47167=CARTESIAN_POINT('Origin',(-53.,19.4,96.)) ;
#47168=CARTESIAN_POINT('',(-52.6,19.4,88.)) ;
#47169=CARTESIAN_POINT('',(-52.6,19.4,96.)) ;
#47170=CARTESIAN_POINT('',(-53.,19.4,88.)) ;
#47171=CARTESIAN_POINT('Origin',(-52.6,19.,96.)) ;
#47172=CARTESIAN_POINT('',(-52.6,19.,88.)) ;
#47173=CARTESIAN_POINT('Origin',(-53.,19.,88.)) ;
#50365=UNCERTAINTY_MEASURE_WITH_UNIT(LENGTH_MEASURE(0.001),#50441,
'DISTANCE_ACCURACY_VALUE',
'Maximum model space distance between geometric entities at asserted c
onnectivities') ;
#50387=UNCERTAINTY_MEASURE_WITH_UNIT(LENGTH_MEASURE(0.001),#50441,
'DISTANCE_ACCURACY_VALUE',
'Maximum model space distance between geometric entities at asserted c
onnectivities') ;
#50418=(
GEOMETRIC_REPRESENTATION_CONTEXT(3)
GLOBAL_UNCERTAINTY_ASSIGNED_CONTEXT((#50365))
GLOBAL_UNIT_ASSIGNED_CONTEXT((#50441,#50443,#50444))
REPRESENTATION_CONTEXT('','3D')
) ;
#50440=(
GEOMETRIC_REPRESENTATION_CONTEXT(3)
GLOBAL_UNCERTAINTY_ASSIGNED_CONTEXT((#50387))
GLOBAL_UNIT_ASSIGNED_CONTEXT((#50441,#50443,#50444))
REPRESENTATION_CONTEXT('','3D')
) ;
#50441=(
LENGTH_UNIT()
NAMED_UNIT(*)
SI_UNIT(.CENTI.,.METRE.)
) ;
#50443=(
NAMED_UNIT(*)
PLANE_ANGLE_UNIT()
SI_UNIT($,.RADIAN.)
) ;
#50444=(
NAMED_UNIT(*)
SI_UNIT($,.STERADIAN.)
SOLID_ANGLE_UNIT()
) ;
#50475=SHAPE_DEFINITION_REPRESENTATION(#50551,#50649) ;
#50551=PRODUCT_DEFINITION_SHAPE('',$,#50702) ;
#50649=SHAPE_REPRESENTATION('',(#30891),#50418) ;
#50671=PRODUCT_DEFINITION_CONTEXT('part definition',#50829,'design') ;
#50702=PRODUCT_DEFINITION('CABLE_ACTUATED_FLOW_CONTROL_LEVER',
'CABLE_ACTUATED_FLOW_CONTROL_LEVER',#50754,#50671) ;
#50754=PRODUCT_DEFINITION_FORMATION('',$,#50861) ;
#50829=APPLICATION_CONTEXT(
'Core Data for Automotive Mechanical Design Process') ;
#50830=PRODUCT_CONTEXT('part definition',#50829,'mechanical') ;
#50861=PRODUCT('CABLE_ACTUATED_FLOW_CONTROL_LEVER',
'CABLE_ACTUATED_FLOW_CONTROL_LEVER',$,(#50830)) ;
#50883=PRESENTATION_STYLE_ASSIGNMENT((#50890)) ;
#50890=SURFACE_STYLE_USAGE(.BOTH.,#50897) ;
#50897=SURFACE_SIDE_STYLE('',(#50904)) ;
#50904=SURFACE_STYLE_FILL_AREA(#50911) ;
#50911=FILL_AREA_STYLE('Steel - Satin',(#50918)) ;
#50918=FILL_AREA_STYLE_COLOUR('Steel - Satin',#50925) ;
#50925=COLOUR_RGB('Steel - Satin', 0.31764706, 0.68627451, 0.89019608) ;
ENDSEC;
END-ISO-10303-21;
